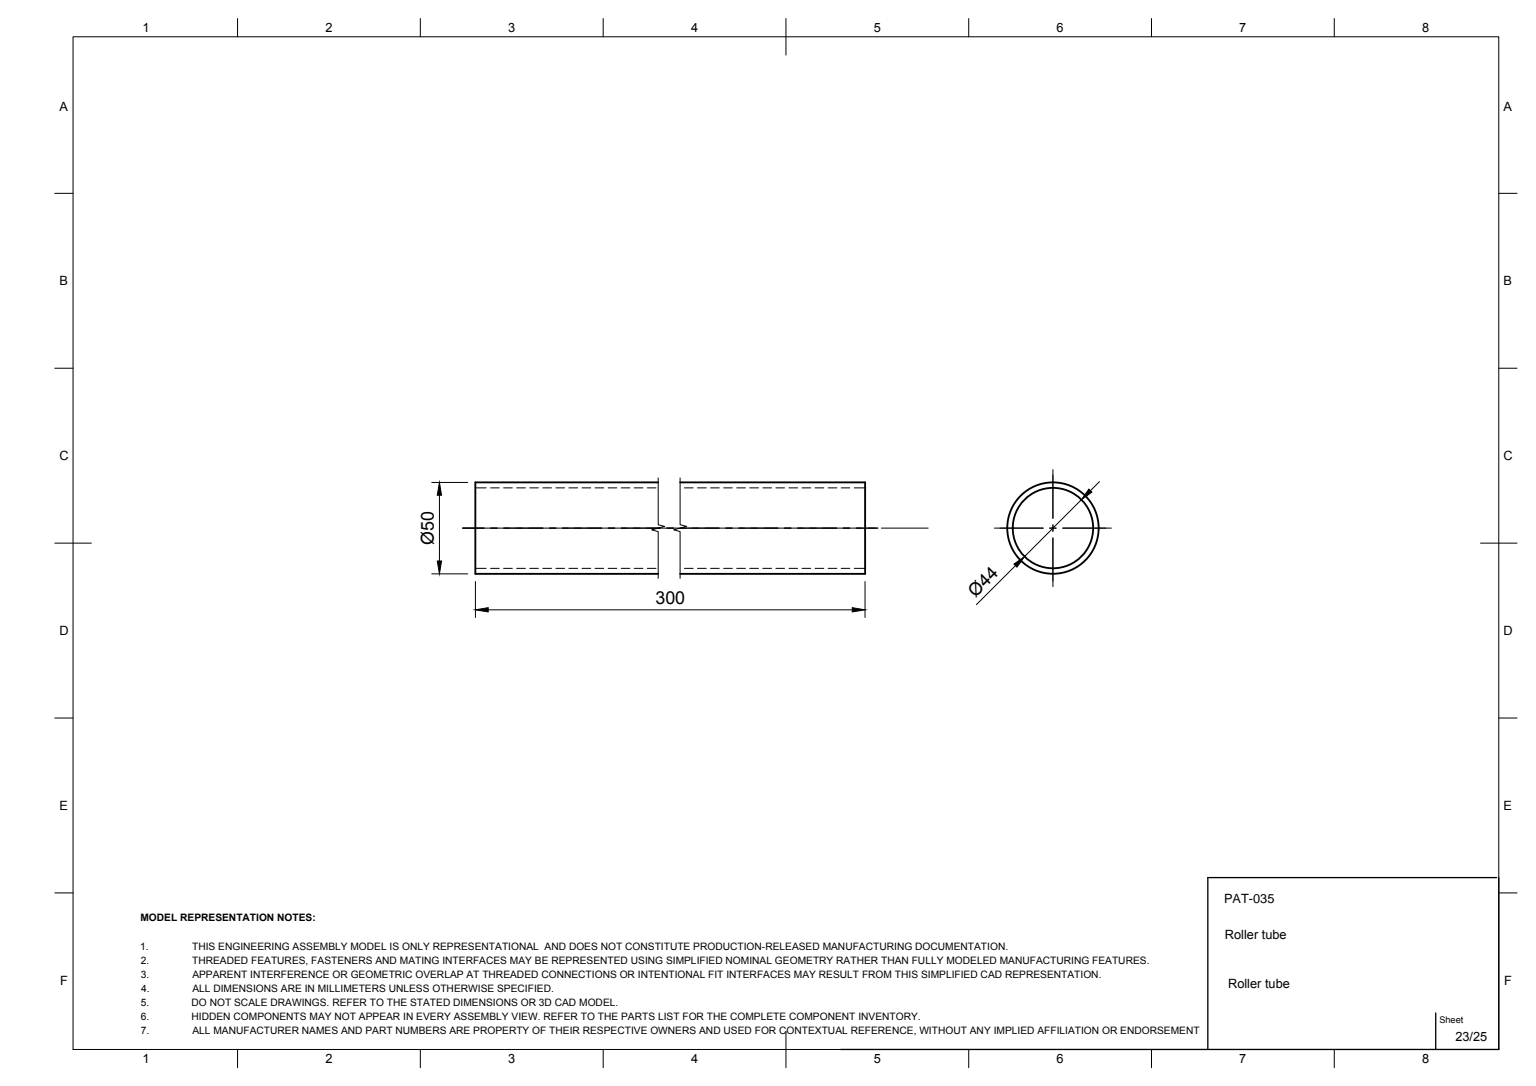
ISO-10303-21;
HEADER;
/* Generated by software containing ST-Developer
 * from STEP Tools, Inc. (www.steptools.com) 
 */

FILE_DESCRIPTION(
/* description */ ('Five-roller gravity conveyor'),
/* implementation_level */ '2;1');

FILE_NAME(
/* name */ 'Roller tube.step',
/* time_stamp */ '2026-10-29T15:36:43-07:00',
/* author */ (''),
/* organization */ (''),
/* preprocessor_version */ 'ST-DEVELOPER v20.2',
/* originating_system */ 'Autodesk Translation Framework v15.17.0.0',
/* authorisation */ '');

FILE_SCHEMA (('AUTOMOTIVE_DESIGN { 1 0 10303 214 3 1 1 }'));
ENDSEC;

DATA;
#10=MECHANICAL_DESIGN_GEOMETRIC_PRESENTATION_REPRESENTATION('',(#334),#7806);
#290=SHAPE_REPRESENTATION_RELATIONSHIP('SRR','None',#7929,#308);
#308=ADVANCED_BREP_SHAPE_REPRESENTATION('',(#359),#7802);
#334=STYLED_ITEM('',(#8077),#359);
#359=MANIFOLD_SOLID_BREP('Body1',#4222);
#397=FACE_BOUND('',#1115,.T.);
#398=FACE_BOUND('',#1117,.T.);
#556=CIRCLE('',#4782,2.2);
#557=CIRCLE('',#4783,2.2);
#558=CIRCLE('',#4785,2.5);
#559=CIRCLE('',#4786,2.5);
#635=CYLINDRICAL_SURFACE('',#4781,2.2);
#636=CYLINDRICAL_SURFACE('',#4784,2.5);
#845=FACE_OUTER_BOUND('',#1112,.T.);
#846=FACE_OUTER_BOUND('',#1113,.T.);
#847=FACE_OUTER_BOUND('',#1114,.T.);
#848=FACE_OUTER_BOUND('',#1116,.T.);
#1112=EDGE_LOOP('',(#3668,#3669,#3670,#3671));
#1113=EDGE_LOOP('',(#3672,#3673,#3674,#3675));
#1114=EDGE_LOOP('',(#3676));
#1115=EDGE_LOOP('',(#3677));
#1116=EDGE_LOOP('',(#3678));
#1117=EDGE_LOOP('',(#3679));
#1477=LINE('',#7546,#1818);
#1478=LINE('',#7552,#1819);
#1818=VECTOR('',#5925,2.2);
#1819=VECTOR('',#5932,2.5);
#2170=VERTEX_POINT('',#7543);
#2171=VERTEX_POINT('',#7545);
#2172=VERTEX_POINT('',#7549);
#2173=VERTEX_POINT('',#7551);
#2677=EDGE_CURVE('',#2170,#2170,#556,.T.);
#2678=EDGE_CURVE('',#2170,#2171,#1477,.T.);
#2679=EDGE_CURVE('',#2171,#2171,#557,.T.);
#2680=EDGE_CURVE('',#2172,#2172,#558,.T.);
#2681=EDGE_CURVE('',#2172,#2173,#1478,.T.);
#2682=EDGE_CURVE('',#2173,#2173,#559,.T.);
#3668=ORIENTED_EDGE('',*,*,#2677,.F.);
#3669=ORIENTED_EDGE('',*,*,#2678,.T.);
#3670=ORIENTED_EDGE('',*,*,#2679,.T.);
#3671=ORIENTED_EDGE('',*,*,#2678,.F.);
#3672=ORIENTED_EDGE('',*,*,#2680,.F.);
#3673=ORIENTED_EDGE('',*,*,#2681,.T.);
#3674=ORIENTED_EDGE('',*,*,#2682,.T.);
#3675=ORIENTED_EDGE('',*,*,#2681,.F.);
#3676=ORIENTED_EDGE('',*,*,#2680,.T.);
#3677=ORIENTED_EDGE('',*,*,#2677,.T.);
#3678=ORIENTED_EDGE('',*,*,#2682,.F.);
#3679=ORIENTED_EDGE('',*,*,#2679,.F.);
#3949=PLANE('',#4787);
#3950=PLANE('',#4788);
#4160=ADVANCED_FACE('',(#845),#635,.F.);
#4161=ADVANCED_FACE('',(#846),#636,.T.);
#4162=ADVANCED_FACE('',(#847,#397),#3949,.T.);
#4163=ADVANCED_FACE('',(#848,#398),#3950,.F.);
#4222=CLOSED_SHELL('',(#4160,#4161,#4162,#4163));
#4780=AXIS2_PLACEMENT_3D('',#7541,#5919,#5920);
#4781=AXIS2_PLACEMENT_3D('',#7542,#5921,#5922);
#4782=AXIS2_PLACEMENT_3D('',#7544,#5923,#5924);
#4783=AXIS2_PLACEMENT_3D('',#7547,#5926,#5927);
#4784=AXIS2_PLACEMENT_3D('',#7548,#5928,#5929);
#4785=AXIS2_PLACEMENT_3D('',#7550,#5930,#5931);
#4786=AXIS2_PLACEMENT_3D('',#7553,#5933,#5934);
#4787=AXIS2_PLACEMENT_3D('',#7554,#5935,#5936);
#4788=AXIS2_PLACEMENT_3D('',#7555,#5937,#5938);
#5919=DIRECTION('axis',(0.,0.,1.));
#5920=DIRECTION('refdir',(1.,0.,0.));
#5921=DIRECTION('center_axis',(0.,1.,0.));
#5922=DIRECTION('ref_axis',(1.,0.,0.));
#5923=DIRECTION('center_axis',(0.,-1.,0.));
#5924=DIRECTION('ref_axis',(1.,0.,0.));
#5925=DIRECTION('',(0.,-1.,0.));
#5926=DIRECTION('center_axis',(0.,-1.,0.));
#5927=DIRECTION('ref_axis',(1.,0.,0.));
#5928=DIRECTION('center_axis',(0.,1.,0.));
#5929=DIRECTION('ref_axis',(1.,0.,0.));
#5930=DIRECTION('center_axis',(0.,1.,0.));
#5931=DIRECTION('ref_axis',(1.,0.,0.));
#5932=DIRECTION('',(0.,-1.,0.));
#5933=DIRECTION('center_axis',(0.,1.,0.));
#5934=DIRECTION('ref_axis',(1.,0.,0.));
#5935=DIRECTION('center_axis',(0.,1.,0.));
#5936=DIRECTION('ref_axis',(1.,0.,0.));
#5937=DIRECTION('center_axis',(0.,1.,0.));
#5938=DIRECTION('ref_axis',(1.,0.,0.));
#7541=CARTESIAN_POINT('',(0.,0.,0.));
#7542=CARTESIAN_POINT('Origin',(0.,0.,4.5));
#7543=CARTESIAN_POINT('',(-2.2,30.,4.5));
#7544=CARTESIAN_POINT('Origin',(0.,30.,4.5));
#7545=CARTESIAN_POINT('',(-2.2,0.,4.5));
#7546=CARTESIAN_POINT('',(-2.2,0.,4.5));
#7547=CARTESIAN_POINT('Origin',(0.,0.,4.5));
#7548=CARTESIAN_POINT('Origin',(0.,0.,4.5));
#7549=CARTESIAN_POINT('',(-2.5,30.,4.5));
#7550=CARTESIAN_POINT('Origin',(0.,30.,4.5));
#7551=CARTESIAN_POINT('',(-2.5,0.,4.5));
#7552=CARTESIAN_POINT('',(-2.5,0.,4.5));
#7553=CARTESIAN_POINT('Origin',(0.,0.,4.5));
#7554=CARTESIAN_POINT('Origin',(0.,30.,4.5));
#7555=CARTESIAN_POINT('Origin',(0.,0.,4.5));
#7778=UNCERTAINTY_MEASURE_WITH_UNIT(LENGTH_MEASURE(0.001),#7807,
'DISTANCE_ACCURACY_VALUE',
'Maximum model space distance between geometric entities at asserted c
onnectivities');
#7782=UNCERTAINTY_MEASURE_WITH_UNIT(LENGTH_MEASURE(0.001),#7807,
'DISTANCE_ACCURACY_VALUE',
'Maximum model space distance between geometric entities at asserted c
onnectivities');
#7802=(
GEOMETRIC_REPRESENTATION_CONTEXT(3)
GLOBAL_UNCERTAINTY_ASSIGNED_CONTEXT((#7778))
GLOBAL_UNIT_ASSIGNED_CONTEXT((#7807,#7809,#7810))
REPRESENTATION_CONTEXT('','3D')
);
#7806=(
GEOMETRIC_REPRESENTATION_CONTEXT(3)
GLOBAL_UNCERTAINTY_ASSIGNED_CONTEXT((#7782))
GLOBAL_UNIT_ASSIGNED_CONTEXT((#7807,#7809,#7810))
REPRESENTATION_CONTEXT('','3D')
);
#7807=(
LENGTH_UNIT()
NAMED_UNIT(*)
SI_UNIT(.CENTI.,.METRE.)
);
#7809=(
NAMED_UNIT(*)
PLANE_ANGLE_UNIT()
SI_UNIT($,.RADIAN.)
);
#7810=(
NAMED_UNIT(*)
SI_UNIT($,.STERADIAN.)
SOLID_ANGLE_UNIT()
);
#7830=SHAPE_DEFINITION_REPRESENTATION(#7858,#7929);
#7858=PRODUCT_DEFINITION_SHAPE('',$,#7953);
#7929=SHAPE_REPRESENTATION('',(#4780),#7802);
#7933=PRODUCT_DEFINITION_CONTEXT('part definition',#8004,'design');
#7953=PRODUCT_DEFINITION('Roller tube','Roller tube',#7976,#7933);
#7976=PRODUCT_DEFINITION_FORMATION('',$,#8025);
#8004=APPLICATION_CONTEXT(
'Core Data for Automotive Mechanical Design Process');
#8005=PRODUCT_CONTEXT('part definition',#8004,'mechanical');
#8025=PRODUCT('Roller tube','Roller tube','Roller tube',(#8005));
#8071=COLOUR_RGB('Light Blue',0.38,0.62,0.78);
#8072=FILL_AREA_STYLE_COLOUR('',#8071);
#8073=FILL_AREA_STYLE('',(#8072));
#8074=SURFACE_STYLE_FILL_AREA(#8073);
#8075=SURFACE_SIDE_STYLE('',(#8074));
#8076=SURFACE_STYLE_USAGE(.BOTH.,#8075);
#8077=PRESENTATION_STYLE_ASSIGNMENT((#8076));
ENDSEC;
END-ISO-10303-21;
